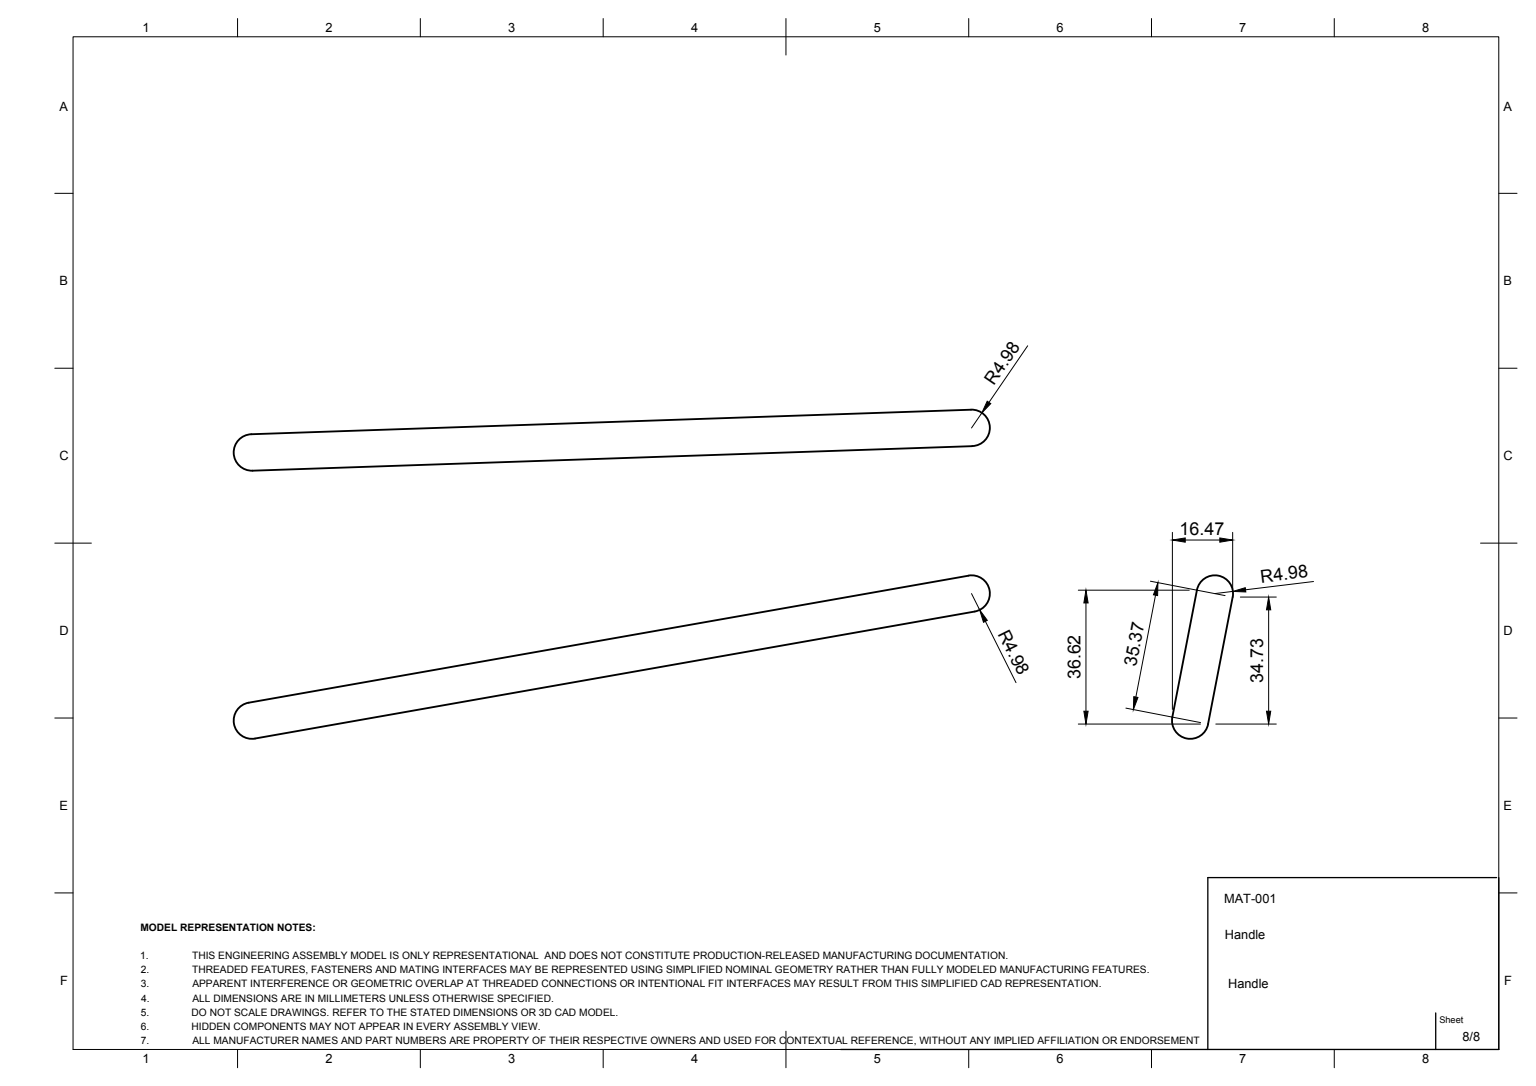
ISO-10303-21;
HEADER;
/* Generated by software containing ST-Developer
 * from STEP Tools, Inc. (www.steptools.com) 
 */

FILE_DESCRIPTION(
/* description */ ('STEP AP214'),
/* implementation_level */ '2;1');

FILE_NAME(
/* name */ 'Handle.step',
/* time_stamp */ '2026-11-14T04:30:00-08:00',
/* author */ (''),
/* organization */ (''),
/* preprocessor_version */ 'ST-DEVELOPER v20.2',
/* originating_system */ 'Autodesk Translation Framework v15.17.0.0',
/* authorisation */ '');

FILE_SCHEMA (('AUTOMOTIVE_DESIGN { 1 0 10303 214 3 1 1 }'));
ENDSEC;

DATA;
#10=MECHANICAL_DESIGN_GEOMETRIC_PRESENTATION_REPRESENTATION('',(#125),#40809);
#109=SHAPE_REPRESENTATION_RELATIONSHIP('SRR','None',#40859,#117);
#117=ADVANCED_BREP_SHAPE_REPRESENTATION('',(#133),#40803);
#125=STYLED_ITEM('',(#40908),#133);
#133=MANIFOLD_SOLID_BREP('Body1',#6300);
#145=SPHERICAL_SURFACE('',#6745,4.975);
#146=SPHERICAL_SURFACE('',#6749,4.975);
#704=FACE_OUTER_BOUND('',#1103,.T.);
#705=FACE_OUTER_BOUND('',#1104,.T.);
#706=FACE_OUTER_BOUND('',#1105,.T.);
#1103=EDGE_LOOP('',(#4920,#4921,#4922,#4923));
#1104=EDGE_LOOP('',(#4924,#4925,#4926,#4927));
#1105=EDGE_LOOP('',(#4928,#4929,#4930,#4931,#4932,#4933));
#1468=CIRCLE('',#6746,4.975);
#1469=CIRCLE('',#6747,4.975);
#1470=CIRCLE('',#6748,4.975);
#1471=CIRCLE('',#6750,4.975);
#1472=CIRCLE('',#6751,4.975);
#1473=CIRCLE('',#6752,4.975);
#1983=LINE('',#39800,#2301);
#2301=VECTOR('',#8059,4.975);
#2757=VERTEX_POINT('',#39786);
#2758=VERTEX_POINT('',#39787);
#2759=VERTEX_POINT('',#39789);
#2760=VERTEX_POINT('',#39793);
#2761=VERTEX_POINT('',#39794);
#2762=VERTEX_POINT('',#39796);
#3512=EDGE_CURVE('',#2757,#2758,#1468,.T.);
#3513=EDGE_CURVE('',#2757,#2759,#1469,.T.);
#3514=EDGE_CURVE('',#2758,#2757,#1470,.T.);
#3515=EDGE_CURVE('',#2760,#2761,#1471,.T.);
#3516=EDGE_CURVE('',#2762,#2761,#1472,.T.);
#3517=EDGE_CURVE('',#2761,#2760,#1473,.T.);
#3518=EDGE_CURVE('',#2758,#2760,#1983,.T.);
#4920=ORIENTED_EDGE('',*,*,#3512,.F.);
#4921=ORIENTED_EDGE('',*,*,#3513,.T.);
#4922=ORIENTED_EDGE('',*,*,#3513,.F.);
#4923=ORIENTED_EDGE('',*,*,#3514,.F.);
#4924=ORIENTED_EDGE('',*,*,#3515,.T.);
#4925=ORIENTED_EDGE('',*,*,#3516,.F.);
#4926=ORIENTED_EDGE('',*,*,#3516,.T.);
#4927=ORIENTED_EDGE('',*,*,#3517,.T.);
#4928=ORIENTED_EDGE('',*,*,#3512,.T.);
#4929=ORIENTED_EDGE('',*,*,#3518,.T.);
#4930=ORIENTED_EDGE('',*,*,#3517,.F.);
#4931=ORIENTED_EDGE('',*,*,#3515,.F.);
#4932=ORIENTED_EDGE('',*,*,#3518,.F.);
#4933=ORIENTED_EDGE('',*,*,#3514,.T.);
#5866=CYLINDRICAL_SURFACE('',#6753,4.975);
#6119=ADVANCED_FACE('',(#704),#145,.T.);
#6120=ADVANCED_FACE('',(#705),#146,.T.);
#6121=ADVANCED_FACE('',(#706),#5866,.T.);
#6300=CLOSED_SHELL('',(#6119,#6120,#6121));
#6744=AXIS2_PLACEMENT_3D('',#39784,#8039,#8040);
#6745=AXIS2_PLACEMENT_3D('',#39785,#8041,#8042);
#6746=AXIS2_PLACEMENT_3D('',#39788,#8043,#8044);
#6747=AXIS2_PLACEMENT_3D('',#39790,#8045,#8046);
#6748=AXIS2_PLACEMENT_3D('',#39791,#8047,#8048);
#6749=AXIS2_PLACEMENT_3D('',#39792,#8049,#8050);
#6750=AXIS2_PLACEMENT_3D('',#39795,#8051,#8052);
#6751=AXIS2_PLACEMENT_3D('',#39797,#8053,#8054);
#6752=AXIS2_PLACEMENT_3D('',#39798,#8055,#8056);
#6753=AXIS2_PLACEMENT_3D('',#39799,#8057,#8058);
#8039=DIRECTION('axis',(0.,0.,1.));
#8040=DIRECTION('refdir',(1.,0.,0.));
#8041=DIRECTION('center_axis',(6.12323399573677E-17,0.,1.));
#8042=DIRECTION('ref_axis',(1.,0.,0.));
#8043=DIRECTION('center_axis',(0.,0.,1.));
#8044=DIRECTION('ref_axis',(1.,0.,0.));
#8045=DIRECTION('center_axis',(1.22464679914735E-16,-1.,0.));
#8046=DIRECTION('ref_axis',(-1.,-1.22464679914735E-16,0.));
#8047=DIRECTION('center_axis',(0.,0.,1.));
#8048=DIRECTION('ref_axis',(1.,0.,0.));
#8049=DIRECTION('center_axis',(6.12323399573677E-17,0.,1.));
#8050=DIRECTION('ref_axis',(1.,0.,0.));
#8051=DIRECTION('center_axis',(0.,0.,1.));
#8052=DIRECTION('ref_axis',(1.,0.,0.));
#8053=DIRECTION('center_axis',(1.22464679914735E-16,-1.,0.));
#8054=DIRECTION('ref_axis',(-1.,-1.22464679914735E-16,0.));
#8055=DIRECTION('center_axis',(0.,0.,1.));
#8056=DIRECTION('ref_axis',(1.,0.,0.));
#8057=DIRECTION('center_axis',(0.,0.,-1.));
#8058=DIRECTION('ref_axis',(-1.,0.,0.));
#8059=DIRECTION('',(0.,0.,1.));
#39784=CARTESIAN_POINT('',(0.,0.,0.));
#39785=CARTESIAN_POINT('Origin',(0.,0.,-100.));
#39786=CARTESIAN_POINT('',(-4.975,0.,-100.));
#39787=CARTESIAN_POINT('',(4.975,-6.09261782575808E-16,-100.));
#39788=CARTESIAN_POINT('Origin',(0.,0.,-100.));
#39789=CARTESIAN_POINT('',(-3.04630891287904E-16,-3.73065245937137E-32,
-104.975));
#39790=CARTESIAN_POINT('Origin',(0.,0.,-100.));
#39791=CARTESIAN_POINT('Origin',(0.,0.,-100.));
#39792=CARTESIAN_POINT('Origin',(0.,0.,100.));
#39793=CARTESIAN_POINT('',(4.975,6.09261782575808E-16,100.));
#39794=CARTESIAN_POINT('',(-4.975,-6.09261782575808E-16,100.));
#39795=CARTESIAN_POINT('Origin',(0.,0.,100.));
#39796=CARTESIAN_POINT('',(-3.04630891287904E-16,-3.73065245937137E-32,
104.975));
#39797=CARTESIAN_POINT('Origin',(0.,0.,100.));
#39798=CARTESIAN_POINT('Origin',(0.,0.,100.));
#39799=CARTESIAN_POINT('Origin',(0.,0.,100.));
#39800=CARTESIAN_POINT('',(4.975,-6.09261782575808E-16,100.));
#40793=UNCERTAINTY_MEASURE_WITH_UNIT(LENGTH_MEASURE(0.01),#40810,
'DISTANCE_ACCURACY_VALUE',
'Maximum model space distance between geometric entities at asserted c
onnectivities');
#40799=UNCERTAINTY_MEASURE_WITH_UNIT(LENGTH_MEASURE(0.01),#40810,
'DISTANCE_ACCURACY_VALUE',
'Maximum model space distance between geometric entities at asserted c
onnectivities');
#40803=(
GEOMETRIC_REPRESENTATION_CONTEXT(3)
GLOBAL_UNCERTAINTY_ASSIGNED_CONTEXT((#40793))
GLOBAL_UNIT_ASSIGNED_CONTEXT((#40810,#40812,#40813))
REPRESENTATION_CONTEXT('','3D')
);
#40809=(
GEOMETRIC_REPRESENTATION_CONTEXT(3)
GLOBAL_UNCERTAINTY_ASSIGNED_CONTEXT((#40799))
GLOBAL_UNIT_ASSIGNED_CONTEXT((#40810,#40812,#40813))
REPRESENTATION_CONTEXT('','3D')
);
#40810=(
LENGTH_UNIT()
NAMED_UNIT(*)
SI_UNIT(.MILLI.,.METRE.)
);
#40812=(
NAMED_UNIT(*)
PLANE_ANGLE_UNIT()
SI_UNIT($,.RADIAN.)
);
#40813=(
NAMED_UNIT(*)
SI_UNIT($,.STERADIAN.)
SOLID_ANGLE_UNIT()
);
#40817=SHAPE_DEFINITION_REPRESENTATION(#40826,#40859);
#40826=PRODUCT_DEFINITION_SHAPE('',$,#40869);
#40859=SHAPE_REPRESENTATION('',(#6744),#40803);
#40865=PRODUCT_DEFINITION_CONTEXT('part definition',#40894,'design');
#40869=PRODUCT_DEFINITION('Handle','Handle',#40878,#40865);
#40878=PRODUCT_DEFINITION_FORMATION('',$,#40899);
#40894=APPLICATION_CONTEXT(
'Core Data for Automotive Mechanical Design Process');
#40895=PRODUCT_CONTEXT('part definition',#40894,'mechanical');
#40899=PRODUCT('Handle','Handle','Handle',(#40895));
#40908=PRESENTATION_STYLE_ASSIGNMENT((#40913));
#40913=SURFACE_STYLE_USAGE(.BOTH.,#40918);
#40918=SURFACE_SIDE_STYLE('',(#40923));
#40923=SURFACE_STYLE_FILL_AREA(#40928);
#40928=FILL_AREA_STYLE('Opaque(61,176,222)',(#40933));
#40933=FILL_AREA_STYLE_COLOUR('Opaque(61,176,222)',#40938);
#40938=COLOUR_RGB('Opaque(61,176,222)',0.23921568627451,0.690196078431373,
0.870588235294118);
ENDSEC;
END-ISO-10303-21;
